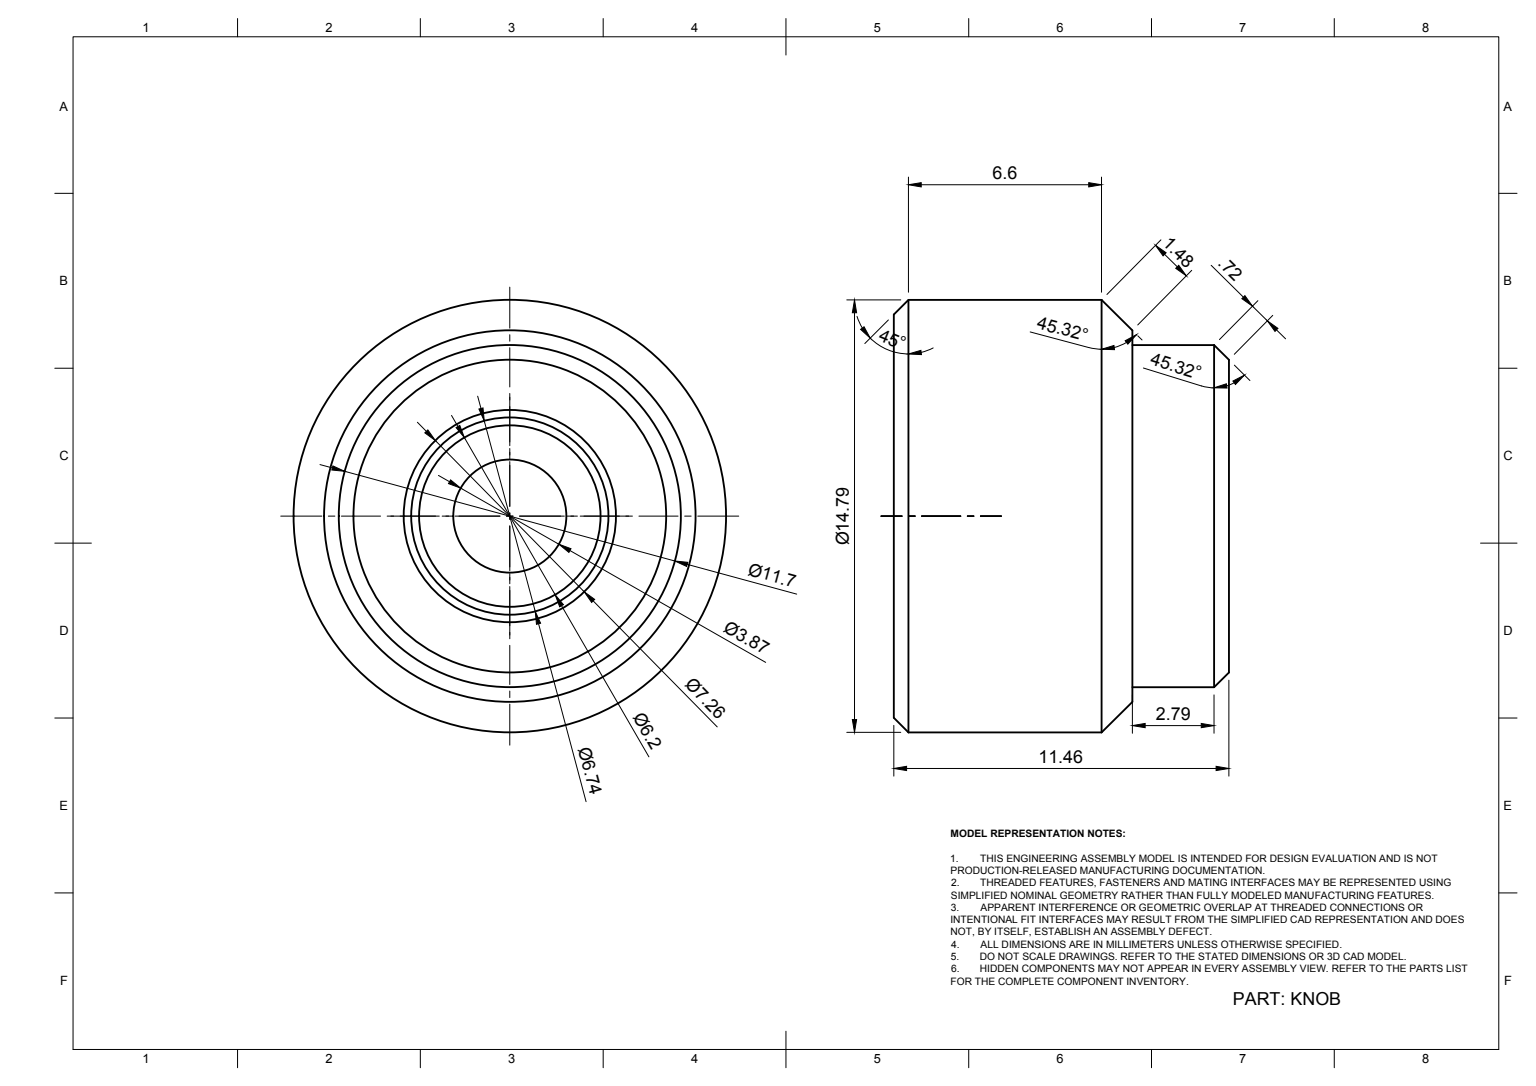
ISO-10303-21;
HEADER;
/* Generated by software containing ST-Developer
 * from STEP Tools, Inc. (www.steptools.com) 
 */

FILE_DESCRIPTION(
/* description */ (''),
/* implementation_level */ '2;1');

FILE_NAME(
/* name */ 'Knob.step',
/* time_stamp */ '2026-10-05T00:51:14-07:00',
/* author */ (''),
/* organization */ (''),
/* preprocessor_version */ 'ST-DEVELOPER v20.2',
/* originating_system */ 'Autodesk Translation Framework v15.15.0.0',
/* authorisation */ '');

FILE_SCHEMA (('AUTOMOTIVE_DESIGN { 1 0 10303 214 3 1 1 }'));
ENDSEC;

DATA;
#10=MECHANICAL_DESIGN_GEOMETRIC_PRESENTATION_REPRESENTATION('',(#389),#4613);
#49=CONICAL_SURFACE('',#1732,7.1427431617401,0.785398163397448);
#50=CONICAL_SURFACE('',#1736,3.05686141031491,0.78225893919059);
#51=CONICAL_SURFACE('',#1750,3.23679059459596,0.791003251258806);
#52=CONICAL_SURFACE('',#1754,3.5004929560726,0.791003251258806);
#53=CONICAL_SURFACE('',#1758,5.5976024439511,0.779793075536092);
#54=CONICAL_SURFACE('',#1764,6.87169679329977,0.779793075536091);
#71=FACE_BOUND('',#534,.T.);
#72=FACE_BOUND('',#537,.T.);
#73=FACE_BOUND('',#540,.T.);
#74=FACE_BOUND('',#543,.T.);
#75=FACE_BOUND('',#549,.T.);
#76=FACE_BOUND('',#553,.T.);
#99=PLANE('',#1734);
#100=PLANE('',#1738);
#101=PLANE('',#1742);
#102=PLANE('',#1746);
#103=PLANE('',#1756);
#104=PLANE('',#1762);
#179=LINE('',#2571,#262);
#180=LINE('',#2575,#263);
#181=LINE('',#2583,#264);
#182=LINE('',#2590,#265);
#183=LINE('',#2597,#266);
#184=LINE('',#2604,#267);
#185=LINE('',#2607,#268);
#186=LINE('',#2612,#269);
#187=LINE('',#2615,#270);
#188=LINE('',#2623,#271);
#189=LINE('',#2627,#272);
#190=LINE('',#2632,#273);
#262=VECTOR('',#1996,7.3927431617401);
#263=VECTOR('',#2001,7.1427431617401);
#264=VECTOR('',#2012,3.05686141031491);
#265=VECTOR('',#2021,1.93367516017024);
#266=VECTOR('',#2030,3.68653879426857);
#267=VECTOR('',#2039,3.10163618786504);
#268=VECTOR('',#2042,3.23679059459596);
#269=VECTOR('',#2049,3.37194500132688);
#270=VECTOR('',#2052,3.5004929560726);
#271=VECTOR('',#2063,5.5976024439511);
#272=VECTOR('',#2068,5.84899819199777);
#273=VECTOR('',#2075,6.87169679329977);
#339=CYLINDRICAL_SURFACE('',#1729,7.3927431617401);
#340=CYLINDRICAL_SURFACE('',#1740,1.93367516017024);
#341=CYLINDRICAL_SURFACE('',#1744,3.68653879426857);
#342=CYLINDRICAL_SURFACE('',#1748,3.10163618786504);
#343=CYLINDRICAL_SURFACE('',#1752,3.37194500132688);
#344=CYLINDRICAL_SURFACE('',#1760,5.84899819199777);
#373=SHAPE_REPRESENTATION_RELATIONSHIP('SRR','None',#4647,#381);
#381=ADVANCED_BREP_SHAPE_REPRESENTATION('',(#397),#4607);
#389=STYLED_ITEM('',(#4696),#397);
#397=MANIFOLD_SOLID_BREP('Body1',#1596);
#421=FACE_OUTER_BOUND('',#531,.T.);
#422=FACE_OUTER_BOUND('',#532,.T.);
#423=FACE_OUTER_BOUND('',#533,.T.);
#424=FACE_OUTER_BOUND('',#535,.T.);
#425=FACE_OUTER_BOUND('',#536,.T.);
#426=FACE_OUTER_BOUND('',#538,.T.);
#427=FACE_OUTER_BOUND('',#539,.T.);
#428=FACE_OUTER_BOUND('',#541,.T.);
#429=FACE_OUTER_BOUND('',#542,.T.);
#430=FACE_OUTER_BOUND('',#544,.T.);
#431=FACE_OUTER_BOUND('',#545,.T.);
#432=FACE_OUTER_BOUND('',#546,.T.);
#433=FACE_OUTER_BOUND('',#547,.T.);
#434=FACE_OUTER_BOUND('',#548,.T.);
#435=FACE_OUTER_BOUND('',#550,.T.);
#436=FACE_OUTER_BOUND('',#551,.T.);
#437=FACE_OUTER_BOUND('',#552,.T.);
#438=FACE_OUTER_BOUND('',#554,.T.);
#531=EDGE_LOOP('',(#1145,#1146,#1147,#1148));
#532=EDGE_LOOP('',(#1149,#1150,#1151,#1152));
#533=EDGE_LOOP('',(#1153));
#534=EDGE_LOOP('',(#1154));
#535=EDGE_LOOP('',(#1155,#1156,#1157,#1158));
#536=EDGE_LOOP('',(#1159));
#537=EDGE_LOOP('',(#1160));
#538=EDGE_LOOP('',(#1161,#1162,#1163,#1164));
#539=EDGE_LOOP('',(#1165));
#540=EDGE_LOOP('',(#1166));
#541=EDGE_LOOP('',(#1167,#1168,#1169,#1170));
#542=EDGE_LOOP('',(#1171));
#543=EDGE_LOOP('',(#1172));
#544=EDGE_LOOP('',(#1173,#1174,#1175,#1176));
#545=EDGE_LOOP('',(#1177,#1178,#1179,#1180));
#546=EDGE_LOOP('',(#1181,#1182,#1183,#1184));
#547=EDGE_LOOP('',(#1185,#1186,#1187,#1188));
#548=EDGE_LOOP('',(#1189));
#549=EDGE_LOOP('',(#1190));
#550=EDGE_LOOP('',(#1191,#1192,#1193,#1194));
#551=EDGE_LOOP('',(#1195,#1196,#1197,#1198));
#552=EDGE_LOOP('',(#1199));
#553=EDGE_LOOP('',(#1200));
#554=EDGE_LOOP('',(#1201,#1202,#1203,#1204));
#655=CIRCLE('',#1730,7.3927431617401);
#656=CIRCLE('',#1731,7.3927431617401);
#657=CIRCLE('',#1733,6.8927431617401);
#658=CIRCLE('',#1735,3.57153586442857);
#659=CIRCLE('',#1737,2.54218695620125);
#660=CIRCLE('',#1739,1.93367516017024);
#661=CIRCLE('',#1741,1.93367516017024);
#662=CIRCLE('',#1743,3.68653879426857);
#663=CIRCLE('',#1745,3.68653879426857);
#664=CIRCLE('',#1747,3.10163618786504);
#665=CIRCLE('',#1749,3.10163618786504);
#666=CIRCLE('',#1751,3.37194500132688);
#667=CIRCLE('',#1753,3.37194500132688);
#668=CIRCLE('',#1755,3.62904091081832);
#669=CIRCLE('',#1757,5.34620669590443);
#670=CIRCLE('',#1759,5.84899819199777);
#671=CIRCLE('',#1761,5.84899819199777);
#672=CIRCLE('',#1763,6.35065042485944);
#756=VERTEX_POINT('',#2568);
#757=VERTEX_POINT('',#2570);
#758=VERTEX_POINT('',#2574);
#759=VERTEX_POINT('',#2578);
#760=VERTEX_POINT('',#2581);
#761=VERTEX_POINT('',#2585);
#762=VERTEX_POINT('',#2588);
#763=VERTEX_POINT('',#2592);
#764=VERTEX_POINT('',#2595);
#765=VERTEX_POINT('',#2599);
#766=VERTEX_POINT('',#2602);
#767=VERTEX_POINT('',#2606);
#768=VERTEX_POINT('',#2610);
#769=VERTEX_POINT('',#2614);
#770=VERTEX_POINT('',#2618);
#771=VERTEX_POINT('',#2621);
#772=VERTEX_POINT('',#2625);
#773=VERTEX_POINT('',#2629);
#900=EDGE_CURVE('',#756,#756,#655,.T.);
#901=EDGE_CURVE('',#756,#757,#179,.T.);
#902=EDGE_CURVE('',#757,#757,#656,.T.);
#903=EDGE_CURVE('',#756,#758,#180,.T.);
#904=EDGE_CURVE('',#758,#758,#657,.T.);
#905=EDGE_CURVE('',#759,#759,#658,.T.);
#906=EDGE_CURVE('',#760,#760,#659,.T.);
#907=EDGE_CURVE('',#760,#759,#181,.T.);
#908=EDGE_CURVE('',#761,#761,#660,.T.);
#909=EDGE_CURVE('',#762,#762,#661,.T.);
#910=EDGE_CURVE('',#762,#761,#182,.T.);
#911=EDGE_CURVE('',#763,#763,#662,.T.);
#912=EDGE_CURVE('',#764,#764,#663,.T.);
#913=EDGE_CURVE('',#764,#763,#183,.T.);
#914=EDGE_CURVE('',#765,#765,#664,.T.);
#915=EDGE_CURVE('',#766,#766,#665,.T.);
#916=EDGE_CURVE('',#766,#765,#184,.T.);
#917=EDGE_CURVE('',#766,#767,#185,.T.);
#918=EDGE_CURVE('',#767,#767,#666,.T.);
#919=EDGE_CURVE('',#768,#768,#667,.T.);
#920=EDGE_CURVE('',#768,#767,#186,.T.);
#921=EDGE_CURVE('',#768,#769,#187,.T.);
#922=EDGE_CURVE('',#769,#769,#668,.T.);
#923=EDGE_CURVE('',#770,#770,#669,.T.);
#924=EDGE_CURVE('',#771,#771,#670,.T.);
#925=EDGE_CURVE('',#771,#770,#188,.T.);
#926=EDGE_CURVE('',#772,#772,#671,.T.);
#927=EDGE_CURVE('',#772,#771,#189,.T.);
#928=EDGE_CURVE('',#773,#773,#672,.T.);
#929=EDGE_CURVE('',#757,#773,#190,.T.);
#1145=ORIENTED_EDGE('',*,*,#900,.F.);
#1146=ORIENTED_EDGE('',*,*,#901,.T.);
#1147=ORIENTED_EDGE('',*,*,#902,.T.);
#1148=ORIENTED_EDGE('',*,*,#901,.F.);
#1149=ORIENTED_EDGE('',*,*,#900,.T.);
#1150=ORIENTED_EDGE('',*,*,#903,.T.);
#1151=ORIENTED_EDGE('',*,*,#904,.F.);
#1152=ORIENTED_EDGE('',*,*,#903,.F.);
#1153=ORIENTED_EDGE('',*,*,#904,.T.);
#1154=ORIENTED_EDGE('',*,*,#905,.F.);
#1155=ORIENTED_EDGE('',*,*,#906,.F.);
#1156=ORIENTED_EDGE('',*,*,#907,.T.);
#1157=ORIENTED_EDGE('',*,*,#905,.T.);
#1158=ORIENTED_EDGE('',*,*,#907,.F.);
#1159=ORIENTED_EDGE('',*,*,#906,.T.);
#1160=ORIENTED_EDGE('',*,*,#908,.F.);
#1161=ORIENTED_EDGE('',*,*,#909,.F.);
#1162=ORIENTED_EDGE('',*,*,#910,.T.);
#1163=ORIENTED_EDGE('',*,*,#908,.T.);
#1164=ORIENTED_EDGE('',*,*,#910,.F.);
#1165=ORIENTED_EDGE('',*,*,#911,.F.);
#1166=ORIENTED_EDGE('',*,*,#909,.T.);
#1167=ORIENTED_EDGE('',*,*,#912,.F.);
#1168=ORIENTED_EDGE('',*,*,#913,.T.);
#1169=ORIENTED_EDGE('',*,*,#911,.T.);
#1170=ORIENTED_EDGE('',*,*,#913,.F.);
#1171=ORIENTED_EDGE('',*,*,#912,.T.);
#1172=ORIENTED_EDGE('',*,*,#914,.F.);
#1173=ORIENTED_EDGE('',*,*,#915,.F.);
#1174=ORIENTED_EDGE('',*,*,#916,.T.);
#1175=ORIENTED_EDGE('',*,*,#914,.T.);
#1176=ORIENTED_EDGE('',*,*,#916,.F.);
#1177=ORIENTED_EDGE('',*,*,#915,.T.);
#1178=ORIENTED_EDGE('',*,*,#917,.T.);
#1179=ORIENTED_EDGE('',*,*,#918,.F.);
#1180=ORIENTED_EDGE('',*,*,#917,.F.);
#1181=ORIENTED_EDGE('',*,*,#919,.F.);
#1182=ORIENTED_EDGE('',*,*,#920,.T.);
#1183=ORIENTED_EDGE('',*,*,#918,.T.);
#1184=ORIENTED_EDGE('',*,*,#920,.F.);
#1185=ORIENTED_EDGE('',*,*,#919,.T.);
#1186=ORIENTED_EDGE('',*,*,#921,.T.);
#1187=ORIENTED_EDGE('',*,*,#922,.F.);
#1188=ORIENTED_EDGE('',*,*,#921,.F.);
#1189=ORIENTED_EDGE('',*,*,#923,.F.);
#1190=ORIENTED_EDGE('',*,*,#922,.T.);
#1191=ORIENTED_EDGE('',*,*,#924,.F.);
#1192=ORIENTED_EDGE('',*,*,#925,.T.);
#1193=ORIENTED_EDGE('',*,*,#923,.T.);
#1194=ORIENTED_EDGE('',*,*,#925,.F.);
#1195=ORIENTED_EDGE('',*,*,#926,.F.);
#1196=ORIENTED_EDGE('',*,*,#927,.T.);
#1197=ORIENTED_EDGE('',*,*,#924,.T.);
#1198=ORIENTED_EDGE('',*,*,#927,.F.);
#1199=ORIENTED_EDGE('',*,*,#928,.F.);
#1200=ORIENTED_EDGE('',*,*,#926,.T.);
#1201=ORIENTED_EDGE('',*,*,#902,.F.);
#1202=ORIENTED_EDGE('',*,*,#929,.T.);
#1203=ORIENTED_EDGE('',*,*,#928,.T.);
#1204=ORIENTED_EDGE('',*,*,#929,.F.);
#1506=ADVANCED_FACE('',(#421),#339,.T.);
#1507=ADVANCED_FACE('',(#422),#49,.T.);
#1508=ADVANCED_FACE('',(#423,#71),#99,.T.);
#1509=ADVANCED_FACE('',(#424),#50,.F.);
#1510=ADVANCED_FACE('',(#425,#72),#100,.T.);
#1511=ADVANCED_FACE('',(#426),#340,.F.);
#1512=ADVANCED_FACE('',(#427,#73),#101,.T.);
#1513=ADVANCED_FACE('',(#428),#341,.F.);
#1514=ADVANCED_FACE('',(#429,#74),#102,.T.);
#1515=ADVANCED_FACE('',(#430),#342,.F.);
#1516=ADVANCED_FACE('',(#431),#51,.F.);
#1517=ADVANCED_FACE('',(#432),#343,.F.);
#1518=ADVANCED_FACE('',(#433),#52,.F.);
#1519=ADVANCED_FACE('',(#434,#75),#103,.T.);
#1520=ADVANCED_FACE('',(#435),#53,.T.);
#1521=ADVANCED_FACE('',(#436),#344,.T.);
#1522=ADVANCED_FACE('',(#437,#76),#104,.T.);
#1523=ADVANCED_FACE('',(#438),#54,.T.);
#1596=CLOSED_SHELL('',(#1506,#1507,#1508,#1509,#1510,#1511,#1512,#1513,
#1514,#1515,#1516,#1517,#1518,#1519,#1520,#1521,#1522,#1523));
#1728=AXIS2_PLACEMENT_3D('',#2566,#1990,#1991);
#1729=AXIS2_PLACEMENT_3D('',#2567,#1992,#1993);
#1730=AXIS2_PLACEMENT_3D('',#2569,#1994,#1995);
#1731=AXIS2_PLACEMENT_3D('',#2572,#1997,#1998);
#1732=AXIS2_PLACEMENT_3D('',#2573,#1999,#2000);
#1733=AXIS2_PLACEMENT_3D('',#2576,#2002,#2003);
#1734=AXIS2_PLACEMENT_3D('',#2577,#2004,#2005);
#1735=AXIS2_PLACEMENT_3D('',#2579,#2006,#2007);
#1736=AXIS2_PLACEMENT_3D('',#2580,#2008,#2009);
#1737=AXIS2_PLACEMENT_3D('',#2582,#2010,#2011);
#1738=AXIS2_PLACEMENT_3D('',#2584,#2013,#2014);
#1739=AXIS2_PLACEMENT_3D('',#2586,#2015,#2016);
#1740=AXIS2_PLACEMENT_3D('',#2587,#2017,#2018);
#1741=AXIS2_PLACEMENT_3D('',#2589,#2019,#2020);
#1742=AXIS2_PLACEMENT_3D('',#2591,#2022,#2023);
#1743=AXIS2_PLACEMENT_3D('',#2593,#2024,#2025);
#1744=AXIS2_PLACEMENT_3D('',#2594,#2026,#2027);
#1745=AXIS2_PLACEMENT_3D('',#2596,#2028,#2029);
#1746=AXIS2_PLACEMENT_3D('',#2598,#2031,#2032);
#1747=AXIS2_PLACEMENT_3D('',#2600,#2033,#2034);
#1748=AXIS2_PLACEMENT_3D('',#2601,#2035,#2036);
#1749=AXIS2_PLACEMENT_3D('',#2603,#2037,#2038);
#1750=AXIS2_PLACEMENT_3D('',#2605,#2040,#2041);
#1751=AXIS2_PLACEMENT_3D('',#2608,#2043,#2044);
#1752=AXIS2_PLACEMENT_3D('',#2609,#2045,#2046);
#1753=AXIS2_PLACEMENT_3D('',#2611,#2047,#2048);
#1754=AXIS2_PLACEMENT_3D('',#2613,#2050,#2051);
#1755=AXIS2_PLACEMENT_3D('',#2616,#2053,#2054);
#1756=AXIS2_PLACEMENT_3D('',#2617,#2055,#2056);
#1757=AXIS2_PLACEMENT_3D('',#2619,#2057,#2058);
#1758=AXIS2_PLACEMENT_3D('',#2620,#2059,#2060);
#1759=AXIS2_PLACEMENT_3D('',#2622,#2061,#2062);
#1760=AXIS2_PLACEMENT_3D('',#2624,#2064,#2065);
#1761=AXIS2_PLACEMENT_3D('',#2626,#2066,#2067);
#1762=AXIS2_PLACEMENT_3D('',#2628,#2069,#2070);
#1763=AXIS2_PLACEMENT_3D('',#2630,#2071,#2072);
#1764=AXIS2_PLACEMENT_3D('',#2631,#2073,#2074);
#1990=DIRECTION('axis',(0.,0.,1.));
#1991=DIRECTION('refdir',(1.,0.,0.));
#1992=DIRECTION('center_axis',(1.,0.,0.));
#1993=DIRECTION('ref_axis',(0.,0.,-1.));
#1994=DIRECTION('center_axis',(1.,0.,0.));
#1995=DIRECTION('ref_axis',(0.,0.,-1.));
#1996=DIRECTION('',(-1.,0.,0.));
#1997=DIRECTION('center_axis',(1.,0.,0.));
#1998=DIRECTION('ref_axis',(0.,0.,-1.));
#1999=DIRECTION('center_axis',(-1.,0.,0.));
#2000=DIRECTION('ref_axis',(0.,0.,-1.));
#2001=DIRECTION('',(0.707106781186548,-8.65956056235493E-17,-0.707106781186547));
#2002=DIRECTION('center_axis',(1.,0.,0.));
#2003=DIRECTION('ref_axis',(0.,0.,-1.));
#2004=DIRECTION('center_axis',(1.,0.,0.));
#2005=DIRECTION('ref_axis',(0.,0.,-1.));
#2006=DIRECTION('center_axis',(1.,0.,0.));
#2007=DIRECTION('ref_axis',(0.,0.,-1.));
#2008=DIRECTION('center_axis',(1.,0.,0.));
#2009=DIRECTION('ref_axis',(0.,0.,-1.));
#2010=DIRECTION('center_axis',(1.,0.,0.));
#2011=DIRECTION('ref_axis',(0.,0.,-1.));
#2012=DIRECTION('',(0.709323060095161,-8.63233363609118E-17,0.704883533938222));
#2013=DIRECTION('center_axis',(1.,0.,0.));
#2014=DIRECTION('ref_axis',(0.,0.,-1.));
#2015=DIRECTION('center_axis',(1.,0.,0.));
#2016=DIRECTION('ref_axis',(0.,0.,-1.));
#2017=DIRECTION('center_axis',(1.,0.,0.));
#2018=DIRECTION('ref_axis',(0.,0.,-1.));
#2019=DIRECTION('center_axis',(1.,0.,0.));
#2020=DIRECTION('ref_axis',(0.,0.,-1.));
#2021=DIRECTION('',(1.,0.,0.));
#2022=DIRECTION('center_axis',(-1.,0.,0.));
#2023=DIRECTION('ref_axis',(0.,0.,1.));
#2024=DIRECTION('center_axis',(1.,0.,0.));
#2025=DIRECTION('ref_axis',(0.,0.,-1.));
#2026=DIRECTION('center_axis',(1.,0.,0.));
#2027=DIRECTION('ref_axis',(0.,0.,-1.));
#2028=DIRECTION('center_axis',(1.,0.,0.));
#2029=DIRECTION('ref_axis',(0.,0.,-1.));
#2030=DIRECTION('',(1.,0.,0.));
#2031=DIRECTION('center_axis',(1.,0.,0.));
#2032=DIRECTION('ref_axis',(0.,0.,-1.));
#2033=DIRECTION('center_axis',(1.,0.,0.));
#2034=DIRECTION('ref_axis',(0.,0.,-1.));
#2035=DIRECTION('center_axis',(1.,0.,0.));
#2036=DIRECTION('ref_axis',(0.,0.,-1.));
#2037=DIRECTION('center_axis',(1.,0.,0.));
#2038=DIRECTION('ref_axis',(0.,0.,-1.));
#2039=DIRECTION('',(1.,0.,0.));
#2040=DIRECTION('center_axis',(-1.,0.,0.));
#2041=DIRECTION('ref_axis',(0.,0.,-1.));
#2042=DIRECTION('',(-0.703132298742306,8.70796187760308E-17,0.711059048508182));
#2043=DIRECTION('center_axis',(1.,0.,0.));
#2044=DIRECTION('ref_axis',(0.,0.,-1.));
#2045=DIRECTION('center_axis',(1.,0.,0.));
#2046=DIRECTION('ref_axis',(0.,0.,-1.));
#2047=DIRECTION('center_axis',(1.,0.,0.));
#2048=DIRECTION('ref_axis',(0.,0.,-1.));
#2049=DIRECTION('',(1.,0.,0.));
#2050=DIRECTION('center_axis',(-1.,0.,0.));
#2051=DIRECTION('ref_axis',(0.,0.,-1.));
#2052=DIRECTION('',(-0.703132298742305,8.70796187760308E-17,0.711059048508182));
#2053=DIRECTION('center_axis',(1.,0.,0.));
#2054=DIRECTION('ref_axis',(0.,0.,-1.));
#2055=DIRECTION('center_axis',(-1.,0.,0.));
#2056=DIRECTION('ref_axis',(0.,0.,1.));
#2057=DIRECTION('center_axis',(1.,0.,0.));
#2058=DIRECTION('ref_axis',(0.,0.,-1.));
#2059=DIRECTION('center_axis',(1.,0.,0.));
#2060=DIRECTION('ref_axis',(0.,0.,-1.));
#2061=DIRECTION('center_axis',(1.,0.,0.));
#2062=DIRECTION('ref_axis',(0.,0.,-1.));
#2063=DIRECTION('',(-0.711059048508181,8.61088719031886E-17,-0.703132298742306));
#2064=DIRECTION('center_axis',(1.,0.,0.));
#2065=DIRECTION('ref_axis',(0.,0.,-1.));
#2066=DIRECTION('center_axis',(1.,0.,0.));
#2067=DIRECTION('ref_axis',(0.,0.,-1.));
#2068=DIRECTION('',(-1.,0.,0.));
#2069=DIRECTION('center_axis',(-1.,0.,0.));
#2070=DIRECTION('ref_axis',(0.,0.,1.));
#2071=DIRECTION('center_axis',(1.,0.,0.));
#2072=DIRECTION('ref_axis',(0.,0.,-1.));
#2073=DIRECTION('center_axis',(1.,0.,0.));
#2074=DIRECTION('ref_axis',(0.,0.,-1.));
#2075=DIRECTION('',(-0.711059048508182,8.61088719031885E-17,-0.703132298742306));
#2566=CARTESIAN_POINT('',(0.,0.,0.));
#2567=CARTESIAN_POINT('Origin',(3.07820337465776,0.,0.));
#2568=CARTESIAN_POINT('',(6.37921955683583,-9.0534992499435E-16,7.3927431617401));
#2569=CARTESIAN_POINT('Origin',(6.37921955683583,0.,0.));
#2570=CARTESIAN_POINT('',(-0.222812807520296,-9.0534992499435E-16,7.3927431617401));
#2571=CARTESIAN_POINT('',(3.07820337465776,-9.0534992499435E-16,7.3927431617401));
#2572=CARTESIAN_POINT('Origin',(-0.222812807520296,0.,0.));
#2573=CARTESIAN_POINT('Origin',(6.62921955683583,0.,0.));
#2574=CARTESIAN_POINT('',(6.87921955683583,-8.44117585036982E-16,6.8927431617401));
#2575=CARTESIAN_POINT('',(6.62921955683583,8.74733755015666E-16,7.1427431617401));
#2576=CARTESIAN_POINT('Origin',(6.87921955683583,0.,0.));
#2577=CARTESIAN_POINT('Origin',(6.87921955683583,0.,-3.57153586442857));
#2578=CARTESIAN_POINT('',(6.87921955683583,-4.37386996441242E-16,3.57153586442857));
#2579=CARTESIAN_POINT('Origin',(6.87921955683583,0.,0.));
#2580=CARTESIAN_POINT('Origin',(6.36130355913187,0.,0.));
#2581=CARTESIAN_POINT('',(5.84338756142791,-3.11328111874601E-16,2.54218695620125));
#2582=CARTESIAN_POINT('Origin',(5.84338756142791,0.,0.));
#2583=CARTESIAN_POINT('',(6.36130355913187,-3.74357554157922E-16,3.05686141031491));
#2584=CARTESIAN_POINT('Origin',(5.84338756142791,0.,-1.93367516017024));
#2585=CARTESIAN_POINT('',(5.84338756142791,-2.36806909549322E-16,1.93367516017024));
#2586=CARTESIAN_POINT('Origin',(5.84338756142791,0.,0.));
#2587=CARTESIAN_POINT('Origin',(2.92894190571765,0.,0.));
#2588=CARTESIAN_POINT('',(0.0144962500073953,-2.36806909549322E-16,1.93367516017024));
#2589=CARTESIAN_POINT('Origin',(0.0144962500073953,0.,0.));
#2590=CARTESIAN_POINT('',(2.92894190571765,-2.36806909549323E-16,1.93367516017024));
#2591=CARTESIAN_POINT('Origin',(0.0144962500073953,0.,-3.68653879426857));
#2592=CARTESIAN_POINT('',(0.0144962500073954,-4.51470793433354E-16,3.68653879426857));
#2593=CARTESIAN_POINT('Origin',(0.0144962500073953,0.,0.));
#2594=CARTESIAN_POINT('Origin',(-0.501553695540098,0.,0.));
#2595=CARTESIAN_POINT('',(-1.01760364108759,-4.51470793433354E-16,3.68653879426857));
#2596=CARTESIAN_POINT('Origin',(-1.01760364108759,0.,0.));
#2597=CARTESIAN_POINT('',(-0.501553695540098,-4.51470793433355E-16,3.68653879426857));
#2598=CARTESIAN_POINT('Origin',(-1.01760364108759,0.,-3.10163618786504));
#2599=CARTESIAN_POINT('',(-1.01760364108759,-3.79840882958852E-16,3.10163618786504));
#2600=CARTESIAN_POINT('Origin',(-1.01760364108759,0.,0.));
#2601=CARTESIAN_POINT('Origin',(-1.65058882961282,0.,0.));
#2602=CARTESIAN_POINT('',(-2.28357401813804,-3.79840882958852E-16,3.10163618786504));
#2603=CARTESIAN_POINT('Origin',(-2.28357401813804,0.,0.));
#2604=CARTESIAN_POINT('',(-1.65058882961282,-3.79840882958852E-16,3.10163618786504));
#2605=CARTESIAN_POINT('Origin',(-2.41722174948925,0.,0.));
#2606=CARTESIAN_POINT('',(-2.55086948084045,-4.12944165277589E-16,3.37194500132688));
#2607=CARTESIAN_POINT('',(-2.41722174948925,3.9639252411822E-16,3.23679059459596));
#2608=CARTESIAN_POINT('Origin',(-2.55086948084045,0.,0.));
#2609=CARTESIAN_POINT('Origin',(-3.43730273109138,0.,0.));
#2610=CARTESIAN_POINT('',(-4.32373598134232,-4.12944165277589E-16,3.37194500132688));
#2611=CARTESIAN_POINT('Origin',(-4.32373598134232,0.,0.));
#2612=CARTESIAN_POINT('',(-3.43730273109138,-4.12944165277588E-16,3.37194500132688));
#2613=CARTESIAN_POINT('Origin',(-4.45085090816676,0.,0.));
#2614=CARTESIAN_POINT('',(-4.57796583499121,-4.44429333540845E-16,3.62904091081832));
#2615=CARTESIAN_POINT('',(-4.45085090816676,4.28686749409217E-16,3.5004929560726));
#2616=CARTESIAN_POINT('Origin',(-4.57796583499121,0.,0.));
#2617=CARTESIAN_POINT('Origin',(-4.57796583499121,0.,-5.34620669590443));
#2618=CARTESIAN_POINT('',(-4.57796583499121,-6.54721491771951E-16,5.34620669590443));
#2619=CARTESIAN_POINT('Origin',(-4.57796583499121,0.,0.));
#2620=CARTESIAN_POINT('Origin',(-4.32373598134232,0.,0.));
#2621=CARTESIAN_POINT('',(-4.06950612769342,-7.16295691404872E-16,5.84899819199777));
#2622=CARTESIAN_POINT('Origin',(-4.06950612769342,0.,0.));
#2623=CARTESIAN_POINT('',(-4.32373598134232,-6.85508591588412E-16,5.5976024439511));
#2624=CARTESIAN_POINT('Origin',(-2.6730798432382,0.,0.));
#2625=CARTESIAN_POINT('',(-1.27665355878298,-7.16295691404872E-16,5.84899819199777));
#2626=CARTESIAN_POINT('Origin',(-1.27665355878298,0.,0.));
#2627=CARTESIAN_POINT('',(-2.6730798432382,-7.16295691404872E-16,5.84899819199777));
#2628=CARTESIAN_POINT('Origin',(-1.27665355878298,0.,-6.35065042485944));
#2629=CARTESIAN_POINT('',(-1.27665355878298,-7.77730371530789E-16,6.35065042485944));
#2630=CARTESIAN_POINT('Origin',(-1.27665355878298,0.,0.));
#2631=CARTESIAN_POINT('Origin',(-0.749733183151639,0.,0.));
#2632=CARTESIAN_POINT('',(-0.749733183151639,-8.41540148262569E-16,6.87169679329977));
#4597=UNCERTAINTY_MEASURE_WITH_UNIT(LENGTH_MEASURE(0.01),#4614,
'DISTANCE_ACCURACY_VALUE',
'Maximum model space distance between geometric entities at asserted c
onnectivities');
#4603=UNCERTAINTY_MEASURE_WITH_UNIT(LENGTH_MEASURE(0.01),#4614,
'DISTANCE_ACCURACY_VALUE',
'Maximum model space distance between geometric entities at asserted c
onnectivities');
#4607=(
GEOMETRIC_REPRESENTATION_CONTEXT(3)
GLOBAL_UNCERTAINTY_ASSIGNED_CONTEXT((#4597))
GLOBAL_UNIT_ASSIGNED_CONTEXT((#4614,#4616,#4617))
REPRESENTATION_CONTEXT('','3D')
);
#4613=(
GEOMETRIC_REPRESENTATION_CONTEXT(3)
GLOBAL_UNCERTAINTY_ASSIGNED_CONTEXT((#4603))
GLOBAL_UNIT_ASSIGNED_CONTEXT((#4614,#4616,#4617))
REPRESENTATION_CONTEXT('','3D')
);
#4614=(
LENGTH_UNIT()
NAMED_UNIT(*)
SI_UNIT(.MILLI.,.METRE.)
);
#4616=(
NAMED_UNIT(*)
PLANE_ANGLE_UNIT()
SI_UNIT($,.RADIAN.)
);
#4617=(
NAMED_UNIT(*)
SI_UNIT($,.STERADIAN.)
SOLID_ANGLE_UNIT()
);
#4621=SHAPE_DEFINITION_REPRESENTATION(#4630,#4647);
#4630=PRODUCT_DEFINITION_SHAPE('',$,#4657);
#4647=SHAPE_REPRESENTATION('',(#1728),#4607);
#4653=PRODUCT_DEFINITION_CONTEXT('part definition',#4682,'design');
#4657=PRODUCT_DEFINITION('Knob','Knob',#4666,#4653);
#4666=PRODUCT_DEFINITION_FORMATION('',$,#4687);
#4682=APPLICATION_CONTEXT(
'Core Data for Automotive Mechanical Design Process');
#4683=PRODUCT_CONTEXT('part definition',#4682,'mechanical');
#4687=PRODUCT('Knob','Knob',$,(#4683));
#4696=PRESENTATION_STYLE_ASSIGNMENT((#4701));
#4701=SURFACE_STYLE_USAGE(.BOTH.,#4706);
#4706=SURFACE_SIDE_STYLE('',(#4711));
#4711=SURFACE_STYLE_FILL_AREA(#4716);
#4716=FILL_AREA_STYLE('Opaque(68,68,68)',(#4721));
#4721=FILL_AREA_STYLE_COLOUR('Opaque(68,68,68)',#4726);
#4726=COLOUR_RGB('Opaque(68,68,68)', 0.31764706, 0.68627451, 0.89019608);
ENDSEC;
END-ISO-10303-21;
